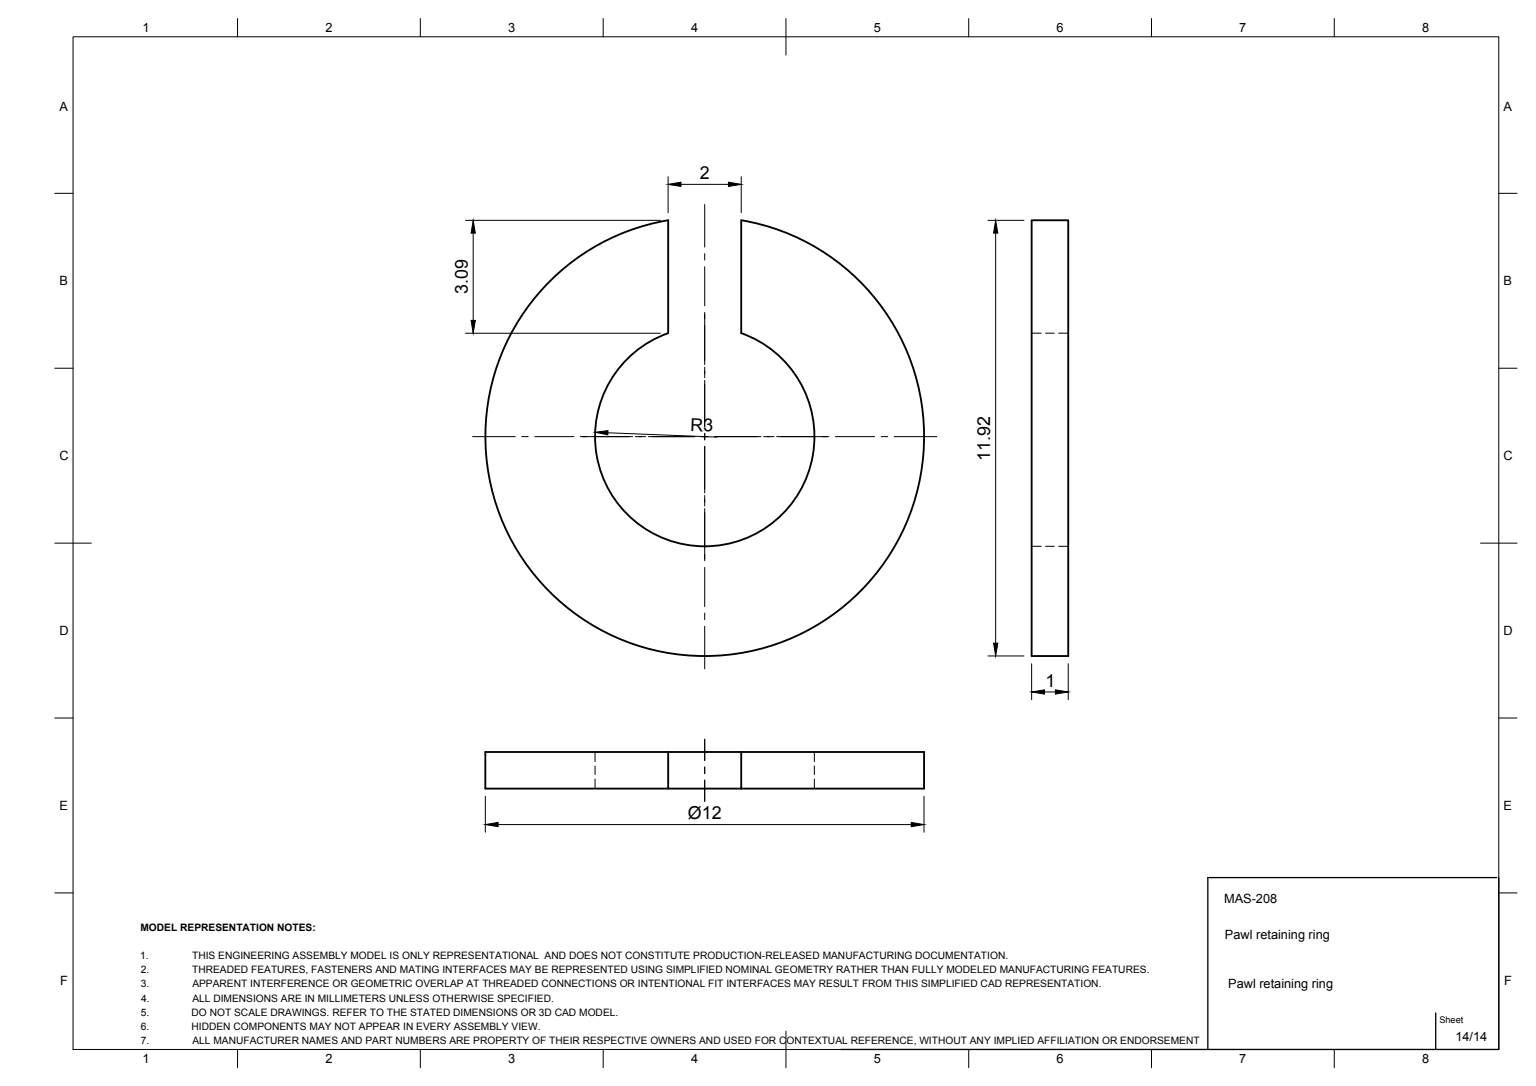
ISO-10303-21;
HEADER;
/* Generated by software containing ST-Developer
 * from STEP Tools, Inc. (www.steptools.com) 
 */

FILE_DESCRIPTION(
/* description */ ('Independent vertical20-tooth ratchet advance with repeated integral-c
ounterweight gravity pawls, swinging drive lever, bronze sleeves and f
ully retained axle stacks.18degpertooth. Native revolutes; geometric c
ycle checking rather than automatic contact/rolling dynamics. Gravity 
closing checked from actual pawl center of mass. Backplate/foot suppor
ts unit. Fits, torque, holding force, wear and life unassigned.'),
/* implementation_level */ '2;1');

FILE_NAME(
/* name */ 'Pawl retaining ring.step',
/* time_stamp */ '2026-11-09T06:25:53-08:00',
/* author */ (''),
/* organization */ (''),
/* preprocessor_version */ 'ST-DEVELOPER v20.2',
/* originating_system */ 'Autodesk Translation Framework v15.17.0.0',
/* authorisation */ '');

FILE_SCHEMA (('AUTOMOTIVE_DESIGN { 1 0 10303 214 3 1 1 }'));
ENDSEC;

DATA;
#10=MECHANICAL_DESIGN_GEOMETRIC_PRESENTATION_REPRESENTATION('',(#136),#4643);
#108=SHAPE_REPRESENTATION_RELATIONSHIP('SRR','None',#4713,#122);
#122=ADVANCED_BREP_SHAPE_REPRESENTATION('',(#150),#4642);
#136=STYLED_ITEM('',(#4783),#150);
#150=MANIFOLD_SOLID_BREP('Body1',#2672);
#300=PLANE('',#3056);
#301=PLANE('',#3057);
#302=PLANE('',#3058);
#303=PLANE('',#3065);
#447=FACE_OUTER_BOUND('',#637,.T.);
#448=FACE_OUTER_BOUND('',#638,.T.);
#449=FACE_OUTER_BOUND('',#639,.T.);
#450=FACE_OUTER_BOUND('',#640,.T.);
#451=FACE_OUTER_BOUND('',#641,.T.);
#452=FACE_OUTER_BOUND('',#642,.T.);
#637=EDGE_LOOP('',(#2449,#2450,#2451,#2452));
#638=EDGE_LOOP('',(#2453,#2454,#2455,#2456));
#639=EDGE_LOOP('',(#2457,#2458,#2459,#2460));
#640=EDGE_LOOP('',(#2461,#2462,#2463,#2464));
#641=EDGE_LOOP('',(#2465,#2466,#2467,#2468));
#642=EDGE_LOOP('',(#2469,#2470,#2471,#2472));
#897=LINE('',#4568,#1159);
#898=LINE('',#4570,#1160);
#899=LINE('',#4572,#1161);
#900=LINE('',#4573,#1162);
#901=LINE('',#4577,#1163);
#902=LINE('',#4579,#1164);
#903=LINE('',#4581,#1165);
#904=LINE('',#4582,#1166);
#1159=VECTOR('',#3799,10.);
#1160=VECTOR('',#3800,10.);
#1161=VECTOR('',#3801,10.);
#1162=VECTOR('',#3802,10.);
#1163=VECTOR('',#3805,10.);
#1164=VECTOR('',#3806,10.);
#1165=VECTOR('',#3807,10.);
#1166=VECTOR('',#3808,10.);
#1237=CIRCLE('',#3059,6.);
#1238=CIRCLE('',#3060,3.);
#1239=CIRCLE('',#3062,3.);
#1240=CIRCLE('',#3064,6.);
#1457=VERTEX_POINT('',#4566);
#1458=VERTEX_POINT('',#4567);
#1459=VERTEX_POINT('',#4569);
#1460=VERTEX_POINT('',#4571);
#1461=VERTEX_POINT('',#4575);
#1462=VERTEX_POINT('',#4576);
#1463=VERTEX_POINT('',#4578);
#1464=VERTEX_POINT('',#4580);
#1789=EDGE_CURVE('',#1457,#1458,#897,.T.);
#1790=EDGE_CURVE('',#1459,#1457,#898,.T.);
#1791=EDGE_CURVE('',#1460,#1459,#899,.T.);
#1792=EDGE_CURVE('',#1458,#1460,#900,.T.);
#1793=EDGE_CURVE('',#1461,#1462,#901,.T.);
#1794=EDGE_CURVE('',#1463,#1461,#902,.T.);
#1795=EDGE_CURVE('',#1464,#1463,#903,.T.);
#1796=EDGE_CURVE('',#1462,#1464,#904,.T.);
#1797=EDGE_CURVE('',#1459,#1464,#1237,.T.);
#1798=EDGE_CURVE('',#1462,#1457,#1238,.T.);
#1799=EDGE_CURVE('',#1461,#1458,#1239,.T.);
#1800=EDGE_CURVE('',#1460,#1463,#1240,.T.);
#2449=ORIENTED_EDGE('',*,*,#1789,.F.);
#2450=ORIENTED_EDGE('',*,*,#1790,.F.);
#2451=ORIENTED_EDGE('',*,*,#1791,.F.);
#2452=ORIENTED_EDGE('',*,*,#1792,.F.);
#2453=ORIENTED_EDGE('',*,*,#1793,.F.);
#2454=ORIENTED_EDGE('',*,*,#1794,.F.);
#2455=ORIENTED_EDGE('',*,*,#1795,.F.);
#2456=ORIENTED_EDGE('',*,*,#1796,.F.);
#2457=ORIENTED_EDGE('',*,*,#1796,.T.);
#2458=ORIENTED_EDGE('',*,*,#1797,.F.);
#2459=ORIENTED_EDGE('',*,*,#1790,.T.);
#2460=ORIENTED_EDGE('',*,*,#1798,.F.);
#2461=ORIENTED_EDGE('',*,*,#1793,.T.);
#2462=ORIENTED_EDGE('',*,*,#1798,.T.);
#2463=ORIENTED_EDGE('',*,*,#1789,.T.);
#2464=ORIENTED_EDGE('',*,*,#1799,.F.);
#2465=ORIENTED_EDGE('',*,*,#1795,.T.);
#2466=ORIENTED_EDGE('',*,*,#1800,.F.);
#2467=ORIENTED_EDGE('',*,*,#1791,.T.);
#2468=ORIENTED_EDGE('',*,*,#1797,.T.);
#2469=ORIENTED_EDGE('',*,*,#1794,.T.);
#2470=ORIENTED_EDGE('',*,*,#1799,.T.);
#2471=ORIENTED_EDGE('',*,*,#1792,.T.);
#2472=ORIENTED_EDGE('',*,*,#1800,.T.);
#2508=CYLINDRICAL_SURFACE('',#3061,3.);
#2509=CYLINDRICAL_SURFACE('',#3063,6.);
#2653=ADVANCED_FACE('',(#447),#300,.F.);
#2654=ADVANCED_FACE('',(#448),#301,.F.);
#2655=ADVANCED_FACE('',(#449),#302,.F.);
#2656=ADVANCED_FACE('',(#450),#2508,.F.);
#2657=ADVANCED_FACE('',(#451),#2509,.T.);
#2658=ADVANCED_FACE('',(#452),#303,.T.);
#2672=CLOSED_SHELL('',(#2653,#2654,#2655,#2656,#2657,#2658));
#3055=AXIS2_PLACEMENT_3D('',#4564,#3795,#3796);
#3056=AXIS2_PLACEMENT_3D('',#4565,#3797,#3798);
#3057=AXIS2_PLACEMENT_3D('',#4574,#3803,#3804);
#3058=AXIS2_PLACEMENT_3D('',#4583,#3809,#3810);
#3059=AXIS2_PLACEMENT_3D('',#4584,#3811,#3812);
#3060=AXIS2_PLACEMENT_3D('',#4585,#3813,#3814);
#3061=AXIS2_PLACEMENT_3D('',#4586,#3815,#3816);
#3062=AXIS2_PLACEMENT_3D('',#4587,#3817,#3818);
#3063=AXIS2_PLACEMENT_3D('',#4588,#3819,#3820);
#3064=AXIS2_PLACEMENT_3D('',#4589,#3821,#3822);
#3065=AXIS2_PLACEMENT_3D('',#4590,#3823,#3824);
#3795=DIRECTION('axis',(0.,0.,1.));
#3796=DIRECTION('refdir',(1.,0.,0.));
#3797=DIRECTION('center_axis',(-1.,0.,0.));
#3798=DIRECTION('ref_axis',(0.,1.,0.));
#3799=DIRECTION('',(0.,0.,1.));
#3800=DIRECTION('',(0.,-1.,0.));
#3801=DIRECTION('',(0.,0.,-1.));
#3802=DIRECTION('',(0.,1.,0.));
#3803=DIRECTION('center_axis',(1.,0.,0.));
#3804=DIRECTION('ref_axis',(0.,-1.,0.));
#3805=DIRECTION('',(0.,0.,-1.));
#3806=DIRECTION('',(0.,-1.,0.));
#3807=DIRECTION('',(0.,0.,1.));
#3808=DIRECTION('',(0.,1.,0.));
#3809=DIRECTION('center_axis',(0.,0.,1.));
#3810=DIRECTION('ref_axis',(1.,0.,0.));
#3811=DIRECTION('center_axis',(0.,0.,1.));
#3812=DIRECTION('ref_axis',(1.,0.,0.));
#3813=DIRECTION('center_axis',(0.,0.,-1.));
#3814=DIRECTION('ref_axis',(1.,0.,0.));
#3815=DIRECTION('center_axis',(0.,0.,1.));
#3816=DIRECTION('ref_axis',(6.12323399573677E-17,-1.,0.));
#3817=DIRECTION('center_axis',(0.,0.,-1.));
#3818=DIRECTION('ref_axis',(1.,0.,0.));
#3819=DIRECTION('center_axis',(0.,0.,1.));
#3820=DIRECTION('ref_axis',(6.12323399573677E-17,-1.,0.));
#3821=DIRECTION('center_axis',(0.,0.,1.));
#3822=DIRECTION('ref_axis',(1.,0.,0.));
#3823=DIRECTION('center_axis',(0.,0.,1.));
#3824=DIRECTION('ref_axis',(1.,0.,0.));
#4564=CARTESIAN_POINT('',(0.,0.,0.));
#4565=CARTESIAN_POINT('Origin',(-1.,0.,1.));
#4566=CARTESIAN_POINT('',(-1.,2.82842712474619,0.));
#4567=CARTESIAN_POINT('',(-1.,2.82842712474619,1.));
#4568=CARTESIAN_POINT('',(-1.,2.82842712474619,0.));
#4569=CARTESIAN_POINT('',(-1.,5.91607978309962,0.));
#4570=CARTESIAN_POINT('',(-1.,0.,0.));
#4571=CARTESIAN_POINT('',(-1.,5.91607978309962,1.));
#4572=CARTESIAN_POINT('',(-1.,5.91607978309962,0.));
#4573=CARTESIAN_POINT('',(-1.,0.,1.));
#4574=CARTESIAN_POINT('Origin',(1.,12.,1.));
#4575=CARTESIAN_POINT('',(1.,2.82842712474619,1.));
#4576=CARTESIAN_POINT('',(1.,2.82842712474619,0.));
#4577=CARTESIAN_POINT('',(1.,2.82842712474619,0.));
#4578=CARTESIAN_POINT('',(1.,5.91607978309962,1.));
#4579=CARTESIAN_POINT('',(1.,6.,1.));
#4580=CARTESIAN_POINT('',(1.,5.91607978309962,0.));
#4581=CARTESIAN_POINT('',(1.,5.91607978309962,0.));
#4582=CARTESIAN_POINT('',(1.,6.,0.));
#4583=CARTESIAN_POINT('Origin',(0.,0.,0.));
#4584=CARTESIAN_POINT('Origin',(0.,0.,0.));
#4585=CARTESIAN_POINT('Origin',(0.,0.,0.));
#4586=CARTESIAN_POINT('Origin',(0.,0.,0.));
#4587=CARTESIAN_POINT('Origin',(0.,0.,1.));
#4588=CARTESIAN_POINT('Origin',(0.,0.,0.));
#4589=CARTESIAN_POINT('Origin',(0.,0.,1.));
#4590=CARTESIAN_POINT('Origin',(0.,0.,1.));
#4626=UNCERTAINTY_MEASURE_WITH_UNIT(LENGTH_MEASURE(0.01),#4644,
'DISTANCE_ACCURACY_VALUE',
'Maximum model space distance between geometric entities at asserted c
onnectivities');
#4627=UNCERTAINTY_MEASURE_WITH_UNIT(LENGTH_MEASURE(0.01),#4644,
'DISTANCE_ACCURACY_VALUE',
'Maximum model space distance between geometric entities at asserted c
onnectivities');
#4642=(
GEOMETRIC_REPRESENTATION_CONTEXT(3)
GLOBAL_UNCERTAINTY_ASSIGNED_CONTEXT((#4626))
GLOBAL_UNIT_ASSIGNED_CONTEXT((#4644,#4646,#4647))
REPRESENTATION_CONTEXT('','3D')
);
#4643=(
GEOMETRIC_REPRESENTATION_CONTEXT(3)
GLOBAL_UNCERTAINTY_ASSIGNED_CONTEXT((#4627))
GLOBAL_UNIT_ASSIGNED_CONTEXT((#4644,#4646,#4647))
REPRESENTATION_CONTEXT('','3D')
);
#4644=(
LENGTH_UNIT()
NAMED_UNIT(*)
SI_UNIT(.MILLI.,.METRE.)
);
#4646=(
NAMED_UNIT(*)
PLANE_ANGLE_UNIT()
SI_UNIT($,.RADIAN.)
);
#4647=(
NAMED_UNIT(*)
SI_UNIT($,.STERADIAN.)
SOLID_ANGLE_UNIT()
);
#4662=SHAPE_DEFINITION_REPRESENTATION(#4677,#4713);
#4677=PRODUCT_DEFINITION_SHAPE('',$,#4729);
#4713=SHAPE_REPRESENTATION('',(#3055),#4642);
#4714=PRODUCT_DEFINITION_CONTEXT('part definition',#4761,'design');
#4729=PRODUCT_DEFINITION('Pawl retaining ring','Pawl retaining ring',#4744,
#4714);
#4744=PRODUCT_DEFINITION_FORMATION('',$,#4777);
#4761=APPLICATION_CONTEXT(
'Core Data for Automotive Mechanical Design Process');
#4762=PRODUCT_CONTEXT('part definition',#4761,'mechanical');
#4777=PRODUCT('Pawl retaining ring','Pawl retaining ring',$,(#4762));
#4783=PRESENTATION_STYLE_ASSIGNMENT((#4792));
#4792=SURFACE_STYLE_USAGE(.BOTH.,#4801);
#4801=SURFACE_SIDE_STYLE('',(#4810));
#4810=SURFACE_STYLE_FILL_AREA(#4819);
#4819=FILL_AREA_STYLE('Dark gray',(#4828));
#4828=FILL_AREA_STYLE_COLOUR('Dark gray',#4837);
#4837=COLOUR_RGB('Dark gray',0.250980392156863,0.282352941176471,0.32156862745098);
ENDSEC;
END-ISO-10303-21;
